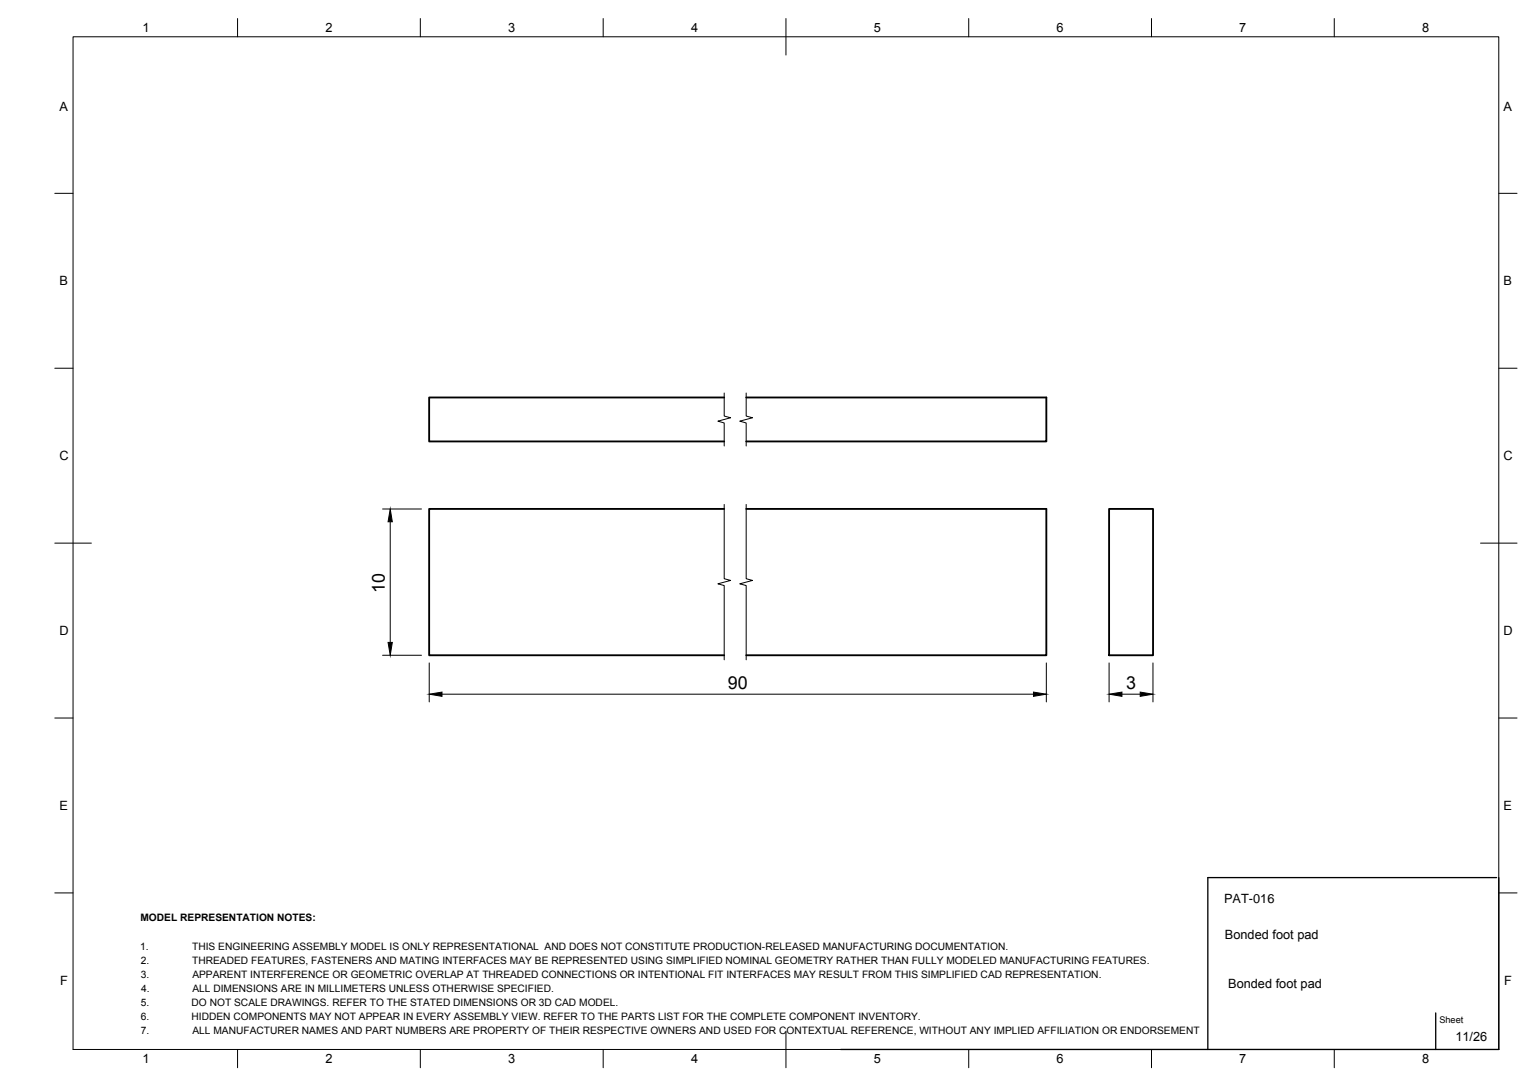
ISO-10303-21;
HEADER;
/* Generated by software containing ST-Developer
 * from STEP Tools, Inc. (www.steptools.com) 
 */

FILE_DESCRIPTION(
/* description */ ('Bracket-mounted idler roller'),
/* implementation_level */ '2;1');

FILE_NAME(
/* name */ 'Bonded foot pad.step',
/* time_stamp */ '2026-10-28T03:26:42-07:00',
/* author */ (''),
/* organization */ (''),
/* preprocessor_version */ 'ST-DEVELOPER v20.2',
/* originating_system */ 'Autodesk Translation Framework v15.17.0.0',
/* authorisation */ '');

FILE_SCHEMA (('AUTOMOTIVE_DESIGN { 1 0 10303 214 3 1 1 }'));
ENDSEC;

DATA;
#10=MECHANICAL_DESIGN_GEOMETRIC_PRESENTATION_REPRESENTATION('',(#286),#6241);
#244=SHAPE_REPRESENTATION_RELATIONSHIP('SRR','None',#6348,#265);
#265=ADVANCED_BREP_SHAPE_REPRESENTATION('',(#315),#6224);
#286=STYLED_ITEM('',(#6531),#315);
#315=MANIFOLD_SOLID_BREP('Body1',#3188);
#455=PLANE('',#3549);
#456=PLANE('',#3550);
#457=PLANE('',#3551);
#458=PLANE('',#3552);
#459=PLANE('',#3553);
#460=PLANE('',#3554);
#573=FACE_OUTER_BOUND('',#794,.T.);
#574=FACE_OUTER_BOUND('',#795,.T.);
#575=FACE_OUTER_BOUND('',#796,.T.);
#576=FACE_OUTER_BOUND('',#797,.T.);
#577=FACE_OUTER_BOUND('',#798,.T.);
#578=FACE_OUTER_BOUND('',#799,.T.);
#794=EDGE_LOOP('',(#2400,#2401,#2402,#2403));
#795=EDGE_LOOP('',(#2404,#2405,#2406,#2407));
#796=EDGE_LOOP('',(#2408,#2409,#2410,#2411));
#797=EDGE_LOOP('',(#2412,#2413,#2414,#2415));
#798=EDGE_LOOP('',(#2416,#2417,#2418,#2419));
#799=EDGE_LOOP('',(#2420,#2421,#2422,#2423));
#1058=LINE('',#5214,#1240);
#1059=LINE('',#5216,#1241);
#1060=LINE('',#5218,#1242);
#1061=LINE('',#5219,#1243);
#1062=LINE('',#5222,#1244);
#1063=LINE('',#5224,#1245);
#1064=LINE('',#5225,#1246);
#1065=LINE('',#5228,#1247);
#1066=LINE('',#5230,#1248);
#1067=LINE('',#5231,#1249);
#1068=LINE('',#5233,#1250);
#1069=LINE('',#5234,#1251);
#1240=VECTOR('',#4175,1.);
#1241=VECTOR('',#4176,1.);
#1242=VECTOR('',#4177,1.);
#1243=VECTOR('',#4178,1.);
#1244=VECTOR('',#4181,1.);
#1245=VECTOR('',#4182,1.);
#1246=VECTOR('',#4183,1.);
#1247=VECTOR('',#4186,1.);
#1248=VECTOR('',#4187,1.);
#1249=VECTOR('',#4188,1.);
#1250=VECTOR('',#4191,1.);
#1251=VECTOR('',#4192,1.);
#1602=VERTEX_POINT('',#5212);
#1603=VERTEX_POINT('',#5213);
#1604=VERTEX_POINT('',#5215);
#1605=VERTEX_POINT('',#5217);
#1606=VERTEX_POINT('',#5221);
#1607=VERTEX_POINT('',#5223);
#1608=VERTEX_POINT('',#5227);
#1609=VERTEX_POINT('',#5229);
#1902=EDGE_CURVE('',#1602,#1603,#1058,.T.);
#1903=EDGE_CURVE('',#1603,#1604,#1059,.T.);
#1904=EDGE_CURVE('',#1605,#1604,#1060,.T.);
#1905=EDGE_CURVE('',#1602,#1605,#1061,.T.);
#1906=EDGE_CURVE('',#1606,#1602,#1062,.T.);
#1907=EDGE_CURVE('',#1607,#1605,#1063,.T.);
#1908=EDGE_CURVE('',#1606,#1607,#1064,.T.);
#1909=EDGE_CURVE('',#1608,#1606,#1065,.T.);
#1910=EDGE_CURVE('',#1609,#1607,#1066,.T.);
#1911=EDGE_CURVE('',#1608,#1609,#1067,.T.);
#1912=EDGE_CURVE('',#1603,#1608,#1068,.T.);
#1913=EDGE_CURVE('',#1604,#1609,#1069,.T.);
#2400=ORIENTED_EDGE('',*,*,#1902,.T.);
#2401=ORIENTED_EDGE('',*,*,#1903,.T.);
#2402=ORIENTED_EDGE('',*,*,#1904,.F.);
#2403=ORIENTED_EDGE('',*,*,#1905,.F.);
#2404=ORIENTED_EDGE('',*,*,#1906,.T.);
#2405=ORIENTED_EDGE('',*,*,#1905,.T.);
#2406=ORIENTED_EDGE('',*,*,#1907,.F.);
#2407=ORIENTED_EDGE('',*,*,#1908,.F.);
#2408=ORIENTED_EDGE('',*,*,#1909,.T.);
#2409=ORIENTED_EDGE('',*,*,#1908,.T.);
#2410=ORIENTED_EDGE('',*,*,#1910,.F.);
#2411=ORIENTED_EDGE('',*,*,#1911,.F.);
#2412=ORIENTED_EDGE('',*,*,#1912,.T.);
#2413=ORIENTED_EDGE('',*,*,#1911,.T.);
#2414=ORIENTED_EDGE('',*,*,#1913,.F.);
#2415=ORIENTED_EDGE('',*,*,#1903,.F.);
#2416=ORIENTED_EDGE('',*,*,#1913,.T.);
#2417=ORIENTED_EDGE('',*,*,#1910,.T.);
#2418=ORIENTED_EDGE('',*,*,#1907,.T.);
#2419=ORIENTED_EDGE('',*,*,#1904,.T.);
#2420=ORIENTED_EDGE('',*,*,#1912,.F.);
#2421=ORIENTED_EDGE('',*,*,#1902,.F.);
#2422=ORIENTED_EDGE('',*,*,#1906,.F.);
#2423=ORIENTED_EDGE('',*,*,#1909,.F.);
#3048=ADVANCED_FACE('',(#573),#455,.T.);
#3049=ADVANCED_FACE('',(#574),#456,.T.);
#3050=ADVANCED_FACE('',(#575),#457,.T.);
#3051=ADVANCED_FACE('',(#576),#458,.T.);
#3052=ADVANCED_FACE('',(#577),#459,.T.);
#3053=ADVANCED_FACE('',(#578),#460,.F.);
#3188=CLOSED_SHELL('',(#3048,#3049,#3050,#3051,#3052,#3053));
#3548=AXIS2_PLACEMENT_3D('',#5210,#4171,#4172);
#3549=AXIS2_PLACEMENT_3D('',#5211,#4173,#4174);
#3550=AXIS2_PLACEMENT_3D('',#5220,#4179,#4180);
#3551=AXIS2_PLACEMENT_3D('',#5226,#4184,#4185);
#3552=AXIS2_PLACEMENT_3D('',#5232,#4189,#4190);
#3553=AXIS2_PLACEMENT_3D('',#5235,#4193,#4194);
#3554=AXIS2_PLACEMENT_3D('',#5236,#4195,#4196);
#4171=DIRECTION('axis',(0.,0.,1.));
#4172=DIRECTION('refdir',(1.,0.,0.));
#4173=DIRECTION('center_axis',(0.,1.,0.));
#4174=DIRECTION('ref_axis',(-1.,0.,0.));
#4175=DIRECTION('',(-1.,0.,0.));
#4176=DIRECTION('',(0.,0.,1.));
#4177=DIRECTION('',(-1.,0.,0.));
#4178=DIRECTION('',(0.,0.,1.));
#4179=DIRECTION('center_axis',(1.,0.,0.));
#4180=DIRECTION('ref_axis',(0.,1.,0.));
#4181=DIRECTION('',(0.,1.,0.));
#4182=DIRECTION('',(0.,1.,0.));
#4183=DIRECTION('',(0.,0.,1.));
#4184=DIRECTION('center_axis',(0.,-1.,0.));
#4185=DIRECTION('ref_axis',(1.,0.,0.));
#4186=DIRECTION('',(1.,0.,0.));
#4187=DIRECTION('',(1.,0.,0.));
#4188=DIRECTION('',(0.,0.,1.));
#4189=DIRECTION('center_axis',(-1.,0.,0.));
#4190=DIRECTION('ref_axis',(0.,-1.,0.));
#4191=DIRECTION('',(0.,-1.,0.));
#4192=DIRECTION('',(0.,-1.,0.));
#4193=DIRECTION('center_axis',(0.,0.,1.));
#4194=DIRECTION('ref_axis',(1.,0.,0.));
#4195=DIRECTION('center_axis',(0.,0.,1.));
#4196=DIRECTION('ref_axis',(1.,0.,0.));
#5210=CARTESIAN_POINT('',(0.,0.,0.));
#5211=CARTESIAN_POINT('Origin',(4.5,-3.,-0.3));
#5212=CARTESIAN_POINT('',(4.5,-3.,-0.3));
#5213=CARTESIAN_POINT('',(-4.5,-3.,-0.3));
#5214=CARTESIAN_POINT('',(4.5,-3.,-0.3));
#5215=CARTESIAN_POINT('',(-4.5,-3.,0.));
#5216=CARTESIAN_POINT('',(-4.5,-3.,-0.3));
#5217=CARTESIAN_POINT('',(4.5,-3.,0.));
#5218=CARTESIAN_POINT('',(4.5,-3.,0.));
#5219=CARTESIAN_POINT('',(4.5,-3.,-0.3));
#5220=CARTESIAN_POINT('Origin',(4.5,-4.,-0.3));
#5221=CARTESIAN_POINT('',(4.5,-4.,-0.3));
#5222=CARTESIAN_POINT('',(4.5,-4.,-0.3));
#5223=CARTESIAN_POINT('',(4.5,-4.,0.));
#5224=CARTESIAN_POINT('',(4.5,-4.,0.));
#5225=CARTESIAN_POINT('',(4.5,-4.,-0.3));
#5226=CARTESIAN_POINT('Origin',(-4.5,-4.,-0.3));
#5227=CARTESIAN_POINT('',(-4.5,-4.,-0.3));
#5228=CARTESIAN_POINT('',(-4.5,-4.,-0.3));
#5229=CARTESIAN_POINT('',(-4.5,-4.,0.));
#5230=CARTESIAN_POINT('',(-4.5,-4.,0.));
#5231=CARTESIAN_POINT('',(-4.5,-4.,-0.3));
#5232=CARTESIAN_POINT('Origin',(-4.5,-3.,-0.3));
#5233=CARTESIAN_POINT('',(-4.5,-3.,-0.3));
#5234=CARTESIAN_POINT('',(-4.5,-3.,0.));
#5235=CARTESIAN_POINT('Origin',(0.,-3.5,0.));
#5236=CARTESIAN_POINT('Origin',(0.,-3.5,-0.3));
#6198=UNCERTAINTY_MEASURE_WITH_UNIT(LENGTH_MEASURE(0.001),#6242,
'DISTANCE_ACCURACY_VALUE',
'Maximum model space distance between geometric entities at asserted c
onnectivities');
#6215=UNCERTAINTY_MEASURE_WITH_UNIT(LENGTH_MEASURE(0.001),#6242,
'DISTANCE_ACCURACY_VALUE',
'Maximum model space distance between geometric entities at asserted c
onnectivities');
#6224=(
GEOMETRIC_REPRESENTATION_CONTEXT(3)
GLOBAL_UNCERTAINTY_ASSIGNED_CONTEXT((#6198))
GLOBAL_UNIT_ASSIGNED_CONTEXT((#6242,#6244,#6245))
REPRESENTATION_CONTEXT('','3D')
);
#6241=(
GEOMETRIC_REPRESENTATION_CONTEXT(3)
GLOBAL_UNCERTAINTY_ASSIGNED_CONTEXT((#6215))
GLOBAL_UNIT_ASSIGNED_CONTEXT((#6242,#6244,#6245))
REPRESENTATION_CONTEXT('','3D')
);
#6242=(
LENGTH_UNIT()
NAMED_UNIT(*)
SI_UNIT(.CENTI.,.METRE.)
);
#6244=(
NAMED_UNIT(*)
PLANE_ANGLE_UNIT()
SI_UNIT($,.RADIAN.)
);
#6245=(
NAMED_UNIT(*)
SI_UNIT($,.STERADIAN.)
SOLID_ANGLE_UNIT()
);
#6254=SHAPE_DEFINITION_REPRESENTATION(#6279,#6348);
#6279=PRODUCT_DEFINITION_SHAPE('',$,#6374);
#6348=SHAPE_REPRESENTATION('',(#3548),#6224);
#6365=PRODUCT_DEFINITION_CONTEXT('part definition',#6442,'design');
#6374=PRODUCT_DEFINITION('Bonded foot pad','Bonded foot pad',#6399,#6365);
#6399=PRODUCT_DEFINITION_FORMATION('',$,#6452);
#6442=APPLICATION_CONTEXT(
'Core Data for Automotive Mechanical Design Process');
#6443=PRODUCT_CONTEXT('part definition',#6442,'mechanical');
#6452=PRODUCT('Bonded foot pad','Bonded foot pad','Bonded foot pad',(#6443));
#6525=COLOUR_RGB('Sky Blue',0.24,0.69,0.87);
#6526=FILL_AREA_STYLE_COLOUR('',#6525);
#6527=FILL_AREA_STYLE('',(#6526));
#6528=SURFACE_STYLE_FILL_AREA(#6527);
#6529=SURFACE_SIDE_STYLE('',(#6528));
#6530=SURFACE_STYLE_USAGE(.BOTH.,#6529);
#6531=PRESENTATION_STYLE_ASSIGNMENT((#6530));
ENDSEC;
END-ISO-10303-21;
